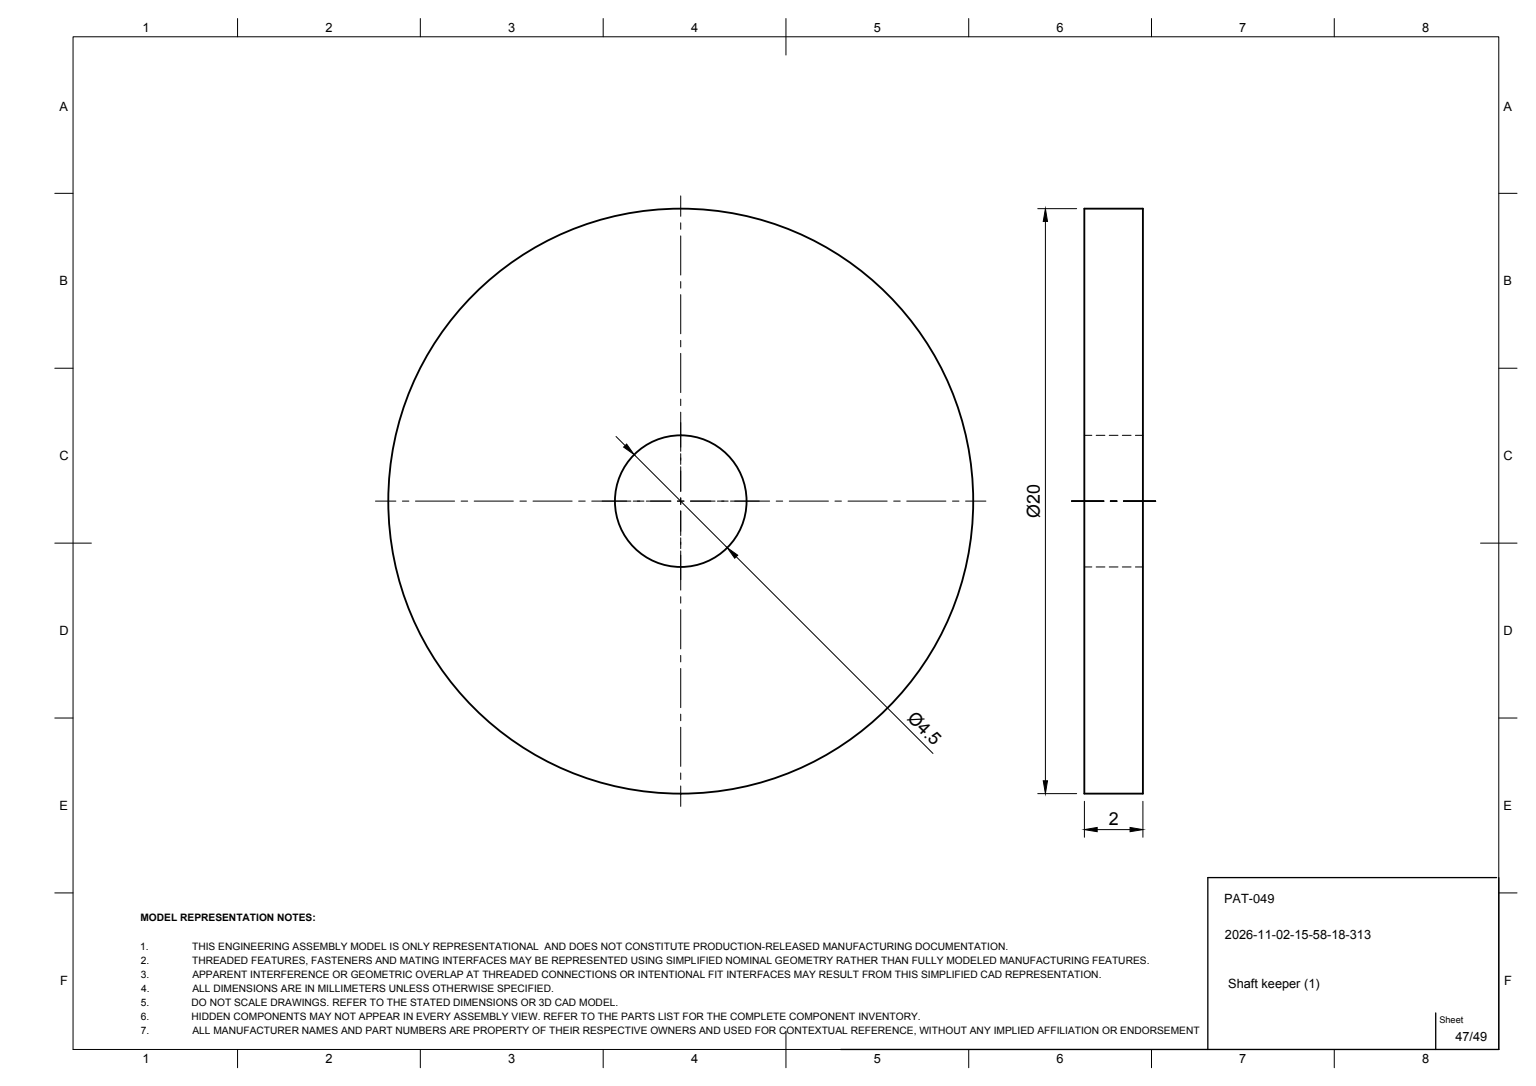
ISO-10303-21;
HEADER;
/* Generated by software containing ST-Developer
 * from STEP Tools, Inc. (www.steptools.com) 
 */

FILE_DESCRIPTION(
/* description */ ('Hand drill press frame (manual)'),
/* implementation_level */ '2;1');

FILE_NAME(
/* name */ 'Shaft keeper (1).step',
/* time_stamp */ '2026-10-28T03:25:28-07:00',
/* author */ (''),
/* organization */ (''),
/* preprocessor_version */ 'ST-DEVELOPER v20.2',
/* originating_system */ 'Autodesk Translation Framework v15.17.0.0',
/* authorisation */ '');

FILE_SCHEMA (('AUTOMOTIVE_DESIGN { 1 0 10303 214 3 1 1 }'));
ENDSEC;

DATA;
#10=MECHANICAL_DESIGN_GEOMETRIC_PRESENTATION_REPRESENTATION('',(#665),#33299);
#568=SHAPE_REPRESENTATION_RELATIONSHIP('SRR','None',#33530,#613);
#613=ADVANCED_BREP_SHAPE_REPRESENTATION('',(#716),#33292);
#665=STYLED_ITEM('',(#33814),#716);
#716=MANIFOLD_SOLID_BREP('Body1',#12684);
#876=FACE_BOUND('',#2742,.T.);
#877=FACE_BOUND('',#2744,.T.);
#1285=PLANE('',#14132);
#1286=PLANE('',#14133);
#1894=FACE_OUTER_BOUND('',#2739,.T.);
#1895=FACE_OUTER_BOUND('',#2740,.T.);
#1896=FACE_OUTER_BOUND('',#2741,.T.);
#1897=FACE_OUTER_BOUND('',#2743,.T.);
#2739=EDGE_LOOP('',(#11111,#11112,#11113,#11114));
#2740=EDGE_LOOP('',(#11115,#11116,#11117,#11118));
#2741=EDGE_LOOP('',(#11119));
#2742=EDGE_LOOP('',(#11120));
#2743=EDGE_LOOP('',(#11121));
#2744=EDGE_LOOP('',(#11122));
#3864=LINE('',#21352,#5029);
#3865=LINE('',#21358,#5030);
#5029=VECTOR('',#17227,0.225);
#5030=VECTOR('',#17234,1.);
#5541=CIRCLE('',#14127,0.225);
#5542=CIRCLE('',#14128,0.225);
#5543=CIRCLE('',#14130,1.);
#5544=CIRCLE('',#14131,1.);
#6517=VERTEX_POINT('',#21349);
#6518=VERTEX_POINT('',#21351);
#6519=VERTEX_POINT('',#21355);
#6520=VERTEX_POINT('',#21357);
#8084=EDGE_CURVE('',#6517,#6517,#5541,.T.);
#8085=EDGE_CURVE('',#6517,#6518,#3864,.T.);
#8086=EDGE_CURVE('',#6518,#6518,#5542,.T.);
#8087=EDGE_CURVE('',#6519,#6519,#5543,.T.);
#8088=EDGE_CURVE('',#6519,#6520,#3865,.T.);
#8089=EDGE_CURVE('',#6520,#6520,#5544,.T.);
#11111=ORIENTED_EDGE('',*,*,#8084,.F.);
#11112=ORIENTED_EDGE('',*,*,#8085,.T.);
#11113=ORIENTED_EDGE('',*,*,#8086,.T.);
#11114=ORIENTED_EDGE('',*,*,#8085,.F.);
#11115=ORIENTED_EDGE('',*,*,#8087,.F.);
#11116=ORIENTED_EDGE('',*,*,#8088,.T.);
#11117=ORIENTED_EDGE('',*,*,#8089,.T.);
#11118=ORIENTED_EDGE('',*,*,#8088,.F.);
#11119=ORIENTED_EDGE('',*,*,#8087,.T.);
#11120=ORIENTED_EDGE('',*,*,#8084,.T.);
#11121=ORIENTED_EDGE('',*,*,#8089,.F.);
#11122=ORIENTED_EDGE('',*,*,#8086,.F.);
#11916=CYLINDRICAL_SURFACE('',#14126,0.225);
#11917=CYLINDRICAL_SURFACE('',#14129,1.);
#12503=ADVANCED_FACE('',(#1894),#11916,.F.);
#12504=ADVANCED_FACE('',(#1895),#11917,.T.);
#12505=ADVANCED_FACE('',(#1896,#876),#1285,.T.);
#12506=ADVANCED_FACE('',(#1897,#877),#1286,.F.);
#12684=CLOSED_SHELL('',(#12503,#12504,#12505,#12506));
#14125=AXIS2_PLACEMENT_3D('',#21347,#17221,#17222);
#14126=AXIS2_PLACEMENT_3D('',#21348,#17223,#17224);
#14127=AXIS2_PLACEMENT_3D('',#21350,#17225,#17226);
#14128=AXIS2_PLACEMENT_3D('',#21353,#17228,#17229);
#14129=AXIS2_PLACEMENT_3D('',#21354,#17230,#17231);
#14130=AXIS2_PLACEMENT_3D('',#21356,#17232,#17233);
#14131=AXIS2_PLACEMENT_3D('',#21359,#17235,#17236);
#14132=AXIS2_PLACEMENT_3D('',#21360,#17237,#17238);
#14133=AXIS2_PLACEMENT_3D('',#21361,#17239,#17240);
#17221=DIRECTION('axis',(0.,0.,1.));
#17222=DIRECTION('refdir',(1.,0.,0.));
#17223=DIRECTION('center_axis',(0.,1.,0.));
#17224=DIRECTION('ref_axis',(1.,0.,0.));
#17225=DIRECTION('center_axis',(0.,-1.,0.));
#17226=DIRECTION('ref_axis',(1.,0.,0.));
#17227=DIRECTION('',(0.,-1.,0.));
#17228=DIRECTION('center_axis',(0.,-1.,0.));
#17229=DIRECTION('ref_axis',(1.,0.,0.));
#17230=DIRECTION('center_axis',(0.,1.,0.));
#17231=DIRECTION('ref_axis',(1.,0.,0.));
#17232=DIRECTION('center_axis',(0.,1.,0.));
#17233=DIRECTION('ref_axis',(1.,0.,0.));
#17234=DIRECTION('',(0.,-1.,0.));
#17235=DIRECTION('center_axis',(0.,1.,0.));
#17236=DIRECTION('ref_axis',(1.,0.,0.));
#17237=DIRECTION('center_axis',(0.,1.,0.));
#17238=DIRECTION('ref_axis',(1.,0.,0.));
#17239=DIRECTION('center_axis',(0.,1.,0.));
#17240=DIRECTION('ref_axis',(1.,0.,0.));
#21347=CARTESIAN_POINT('',(0.,0.,0.));
#21348=CARTESIAN_POINT('Origin',(-3.25,7.5,20.));
#21349=CARTESIAN_POINT('',(-3.475,7.7,20.));
#21350=CARTESIAN_POINT('Origin',(-3.25,7.7,20.));
#21351=CARTESIAN_POINT('',(-3.475,7.5,20.));
#21352=CARTESIAN_POINT('',(-3.475,7.5,20.));
#21353=CARTESIAN_POINT('Origin',(-3.25,7.5,20.));
#21354=CARTESIAN_POINT('Origin',(-3.25,7.5,20.));
#21355=CARTESIAN_POINT('',(-4.25,7.7,20.));
#21356=CARTESIAN_POINT('Origin',(-3.25,7.7,20.));
#21357=CARTESIAN_POINT('',(-4.25,7.5,20.));
#21358=CARTESIAN_POINT('',(-4.25,7.5,20.));
#21359=CARTESIAN_POINT('Origin',(-3.25,7.5,20.));
#21360=CARTESIAN_POINT('Origin',(-3.25,7.7,20.));
#21361=CARTESIAN_POINT('Origin',(-3.25,7.5,20.));
#33240=UNCERTAINTY_MEASURE_WITH_UNIT(LENGTH_MEASURE(0.001),#33300,
'DISTANCE_ACCURACY_VALUE',
'Maximum model space distance between geometric entities at asserted c
onnectivities');
#33247=UNCERTAINTY_MEASURE_WITH_UNIT(LENGTH_MEASURE(0.001),#33300,
'DISTANCE_ACCURACY_VALUE',
'Maximum model space distance between geometric entities at asserted c
onnectivities');
#33292=(
GEOMETRIC_REPRESENTATION_CONTEXT(3)
GLOBAL_UNCERTAINTY_ASSIGNED_CONTEXT((#33240))
GLOBAL_UNIT_ASSIGNED_CONTEXT((#33300,#33302,#33303))
REPRESENTATION_CONTEXT('','3D')
);
#33299=(
GEOMETRIC_REPRESENTATION_CONTEXT(3)
GLOBAL_UNCERTAINTY_ASSIGNED_CONTEXT((#33247))
GLOBAL_UNIT_ASSIGNED_CONTEXT((#33300,#33302,#33303))
REPRESENTATION_CONTEXT('','3D')
);
#33300=(
LENGTH_UNIT()
NAMED_UNIT(*)
SI_UNIT(.CENTI.,.METRE.)
);
#33302=(
NAMED_UNIT(*)
PLANE_ANGLE_UNIT()
SI_UNIT($,.RADIAN.)
);
#33303=(
NAMED_UNIT(*)
SI_UNIT($,.STERADIAN.)
SOLID_ANGLE_UNIT()
);
#33348=SHAPE_DEFINITION_REPRESENTATION(#33410,#33530);
#33410=PRODUCT_DEFINITION_SHAPE('',$,#33582);
#33530=SHAPE_REPRESENTATION('',(#14125),#33292);
#33537=PRODUCT_DEFINITION_CONTEXT('part definition',#33692,'design');
#33582=PRODUCT_DEFINITION('Shaft keeper (1)','Shaft keeper (1)',#33633,#33537);
#33633=PRODUCT_DEFINITION_FORMATION('',$,#33738);
#33692=APPLICATION_CONTEXT(
'Core Data for Automotive Mechanical Design Process');
#33693=PRODUCT_CONTEXT('part definition',#33692,'mechanical');
#33738=PRODUCT('Shaft keeper (1)','Shaft keeper (1)','Shaft keeper (1)',(#33693));
#33808=COLOUR_RGB('Grey',0.48,0.52,0.57);
#33809=FILL_AREA_STYLE_COLOUR('',#33808);
#33810=FILL_AREA_STYLE('',(#33809));
#33811=SURFACE_STYLE_FILL_AREA(#33810);
#33812=SURFACE_SIDE_STYLE('',(#33811));
#33813=SURFACE_STYLE_USAGE(.BOTH.,#33812);
#33814=PRESENTATION_STYLE_ASSIGNMENT((#33813));
ENDSEC;
END-ISO-10303-21;
